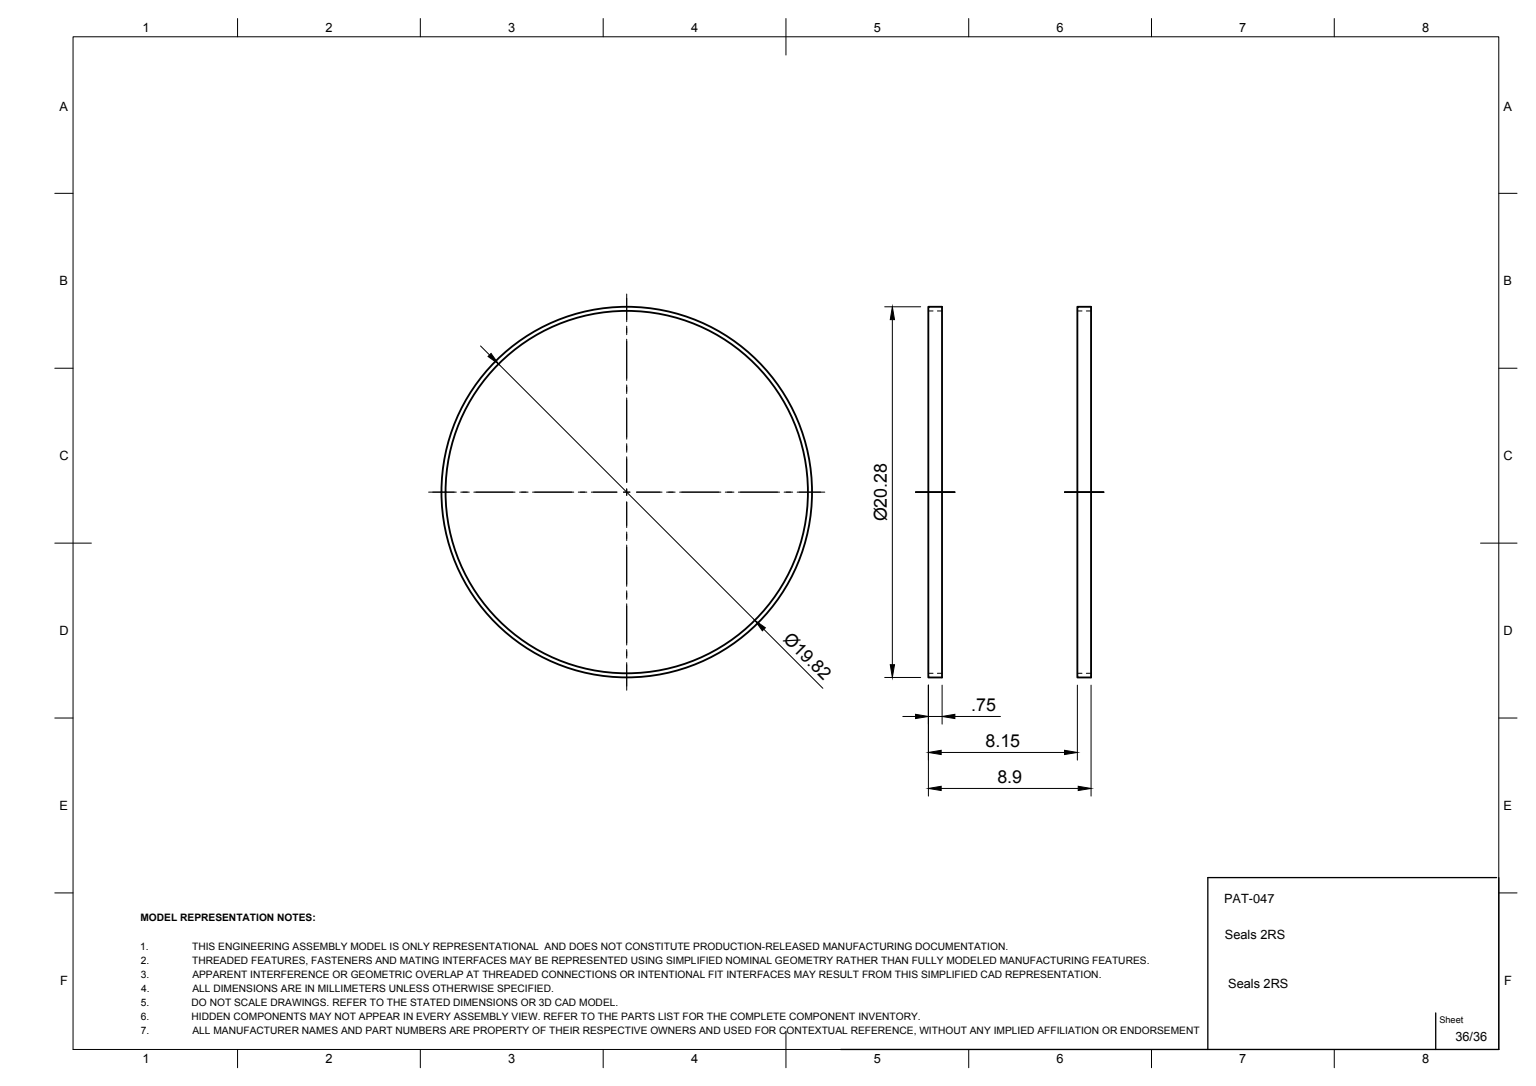
ISO-10303-21;
HEADER;
/* Generated by software containing ST-Developer
 * from STEP Tools, Inc. (www.steptools.com) 
 */

FILE_DESCRIPTION(
/* description */ ('Gravity roller conveyor section'),
/* implementation_level */ '2;1');

FILE_NAME(
/* name */ 'Seals 2RS.step',
/* time_stamp */ '2026-11-02T07:43:02-08:00',
/* author */ (''),
/* organization */ (''),
/* preprocessor_version */ 'ST-DEVELOPER v20.2',
/* originating_system */ 'Autodesk Translation Framework v15.17.0.0',
/* authorisation */ '');

FILE_SCHEMA (('AUTOMOTIVE_DESIGN { 1 0 10303 214 3 1 1 }'));
ENDSEC;

DATA;
#10=MECHANICAL_DESIGN_GEOMETRIC_PRESENTATION_REPRESENTATION('',(#563,#564),#13821);
#488=SHAPE_REPRESENTATION_RELATIONSHIP('SRR','None',#14027,#522);
#522=ADVANCED_BREP_SHAPE_REPRESENTATION('',(#603,#604),#13814);
#563=STYLED_ITEM('',(#14192),#603);
#564=STYLED_ITEM('',(#14192),#604);
#603=MANIFOLD_SOLID_BREP('Body1',#7663);
#604=MANIFOLD_SOLID_BREP('Body2',#7664);
#683=FACE_BOUND('',#1845,.T.);
#684=FACE_BOUND('',#1848,.T.);
#685=FACE_BOUND('',#1851,.T.);
#686=FACE_BOUND('',#1854,.T.);
#956=PLANE('',#8596);
#957=PLANE('',#8601);
#958=PLANE('',#8604);
#959=PLANE('',#8609);
#1351=FACE_OUTER_BOUND('',#1844,.T.);
#1352=FACE_OUTER_BOUND('',#1846,.T.);
#1353=FACE_OUTER_BOUND('',#1847,.T.);
#1354=FACE_OUTER_BOUND('',#1849,.T.);
#1355=FACE_OUTER_BOUND('',#1850,.T.);
#1356=FACE_OUTER_BOUND('',#1852,.T.);
#1357=FACE_OUTER_BOUND('',#1853,.T.);
#1358=FACE_OUTER_BOUND('',#1855,.T.);
#1844=EDGE_LOOP('',(#6830));
#1845=EDGE_LOOP('',(#6831));
#1846=EDGE_LOOP('',(#6832,#6833,#6834,#6835));
#1847=EDGE_LOOP('',(#6836));
#1848=EDGE_LOOP('',(#6837));
#1849=EDGE_LOOP('',(#6838,#6839,#6840,#6841));
#1850=EDGE_LOOP('',(#6842));
#1851=EDGE_LOOP('',(#6843));
#1852=EDGE_LOOP('',(#6844,#6845,#6846,#6847));
#1853=EDGE_LOOP('',(#6848));
#1854=EDGE_LOOP('',(#6849));
#1855=EDGE_LOOP('',(#6850,#6851,#6852,#6853));
#2552=LINE('',#13329,#3270);
#2553=LINE('',#13334,#3271);
#2554=LINE('',#13343,#3272);
#2555=LINE('',#13348,#3273);
#3270=VECTOR('',#10537,1.013815);
#3271=VECTOR('',#10544,0.991185);
#3272=VECTOR('',#10555,1.013815);
#3273=VECTOR('',#10562,0.991185);
#3546=CIRCLE('',#8597,1.013815);
#3547=CIRCLE('',#8598,0.991185);
#3548=CIRCLE('',#8600,1.013815);
#3549=CIRCLE('',#8602,0.991185);
#3550=CIRCLE('',#8605,1.013815);
#3551=CIRCLE('',#8606,0.991185);
#3552=CIRCLE('',#8608,1.013815);
#3553=CIRCLE('',#8610,0.991185);
#4140=VERTEX_POINT('',#13322);
#4141=VERTEX_POINT('',#13324);
#4142=VERTEX_POINT('',#13327);
#4143=VERTEX_POINT('',#13331);
#4144=VERTEX_POINT('',#13336);
#4145=VERTEX_POINT('',#13338);
#4146=VERTEX_POINT('',#13341);
#4147=VERTEX_POINT('',#13345);
#5052=EDGE_CURVE('',#4140,#4140,#3546,.T.);
#5053=EDGE_CURVE('',#4141,#4141,#3547,.T.);
#5054=EDGE_CURVE('',#4142,#4142,#3548,.T.);
#5055=EDGE_CURVE('',#4142,#4140,#2552,.T.);
#5056=EDGE_CURVE('',#4143,#4143,#3549,.T.);
#5057=EDGE_CURVE('',#4143,#4141,#2553,.T.);
#5058=EDGE_CURVE('',#4144,#4144,#3550,.T.);
#5059=EDGE_CURVE('',#4145,#4145,#3551,.T.);
#5060=EDGE_CURVE('',#4146,#4146,#3552,.T.);
#5061=EDGE_CURVE('',#4146,#4144,#2554,.T.);
#5062=EDGE_CURVE('',#4147,#4147,#3553,.T.);
#5063=EDGE_CURVE('',#4147,#4145,#2555,.T.);
#6830=ORIENTED_EDGE('',*,*,#5052,.F.);
#6831=ORIENTED_EDGE('',*,*,#5053,.T.);
#6832=ORIENTED_EDGE('',*,*,#5054,.F.);
#6833=ORIENTED_EDGE('',*,*,#5055,.T.);
#6834=ORIENTED_EDGE('',*,*,#5052,.T.);
#6835=ORIENTED_EDGE('',*,*,#5055,.F.);
#6836=ORIENTED_EDGE('',*,*,#5054,.T.);
#6837=ORIENTED_EDGE('',*,*,#5056,.F.);
#6838=ORIENTED_EDGE('',*,*,#5056,.T.);
#6839=ORIENTED_EDGE('',*,*,#5057,.T.);
#6840=ORIENTED_EDGE('',*,*,#5053,.F.);
#6841=ORIENTED_EDGE('',*,*,#5057,.F.);
#6842=ORIENTED_EDGE('',*,*,#5058,.F.);
#6843=ORIENTED_EDGE('',*,*,#5059,.T.);
#6844=ORIENTED_EDGE('',*,*,#5060,.F.);
#6845=ORIENTED_EDGE('',*,*,#5061,.T.);
#6846=ORIENTED_EDGE('',*,*,#5058,.T.);
#6847=ORIENTED_EDGE('',*,*,#5061,.F.);
#6848=ORIENTED_EDGE('',*,*,#5060,.T.);
#6849=ORIENTED_EDGE('',*,*,#5062,.F.);
#6850=ORIENTED_EDGE('',*,*,#5062,.T.);
#6851=ORIENTED_EDGE('',*,*,#5063,.T.);
#6852=ORIENTED_EDGE('',*,*,#5059,.F.);
#6853=ORIENTED_EDGE('',*,*,#5063,.F.);
#7190=CYLINDRICAL_SURFACE('',#8599,1.013815);
#7191=CYLINDRICAL_SURFACE('',#8603,0.991185);
#7192=CYLINDRICAL_SURFACE('',#8607,1.013815);
#7193=CYLINDRICAL_SURFACE('',#8611,0.991185);
#7552=ADVANCED_FACE('',(#1351,#683),#956,.T.);
#7553=ADVANCED_FACE('',(#1352),#7190,.T.);
#7554=ADVANCED_FACE('',(#1353,#684),#957,.T.);
#7555=ADVANCED_FACE('',(#1354),#7191,.F.);
#7556=ADVANCED_FACE('',(#1355,#685),#958,.T.);
#7557=ADVANCED_FACE('',(#1356),#7192,.T.);
#7558=ADVANCED_FACE('',(#1357,#686),#959,.T.);
#7559=ADVANCED_FACE('',(#1358),#7193,.F.);
#7663=CLOSED_SHELL('',(#7552,#7553,#7554,#7555));
#7664=CLOSED_SHELL('',(#7556,#7557,#7558,#7559));
#8595=AXIS2_PLACEMENT_3D('',#13320,#10525,#10526);
#8596=AXIS2_PLACEMENT_3D('',#13321,#10527,#10528);
#8597=AXIS2_PLACEMENT_3D('',#13323,#10529,#10530);
#8598=AXIS2_PLACEMENT_3D('',#13325,#10531,#10532);
#8599=AXIS2_PLACEMENT_3D('',#13326,#10533,#10534);
#8600=AXIS2_PLACEMENT_3D('',#13328,#10535,#10536);
#8601=AXIS2_PLACEMENT_3D('',#13330,#10538,#10539);
#8602=AXIS2_PLACEMENT_3D('',#13332,#10540,#10541);
#8603=AXIS2_PLACEMENT_3D('',#13333,#10542,#10543);
#8604=AXIS2_PLACEMENT_3D('',#13335,#10545,#10546);
#8605=AXIS2_PLACEMENT_3D('',#13337,#10547,#10548);
#8606=AXIS2_PLACEMENT_3D('',#13339,#10549,#10550);
#8607=AXIS2_PLACEMENT_3D('',#13340,#10551,#10552);
#8608=AXIS2_PLACEMENT_3D('',#13342,#10553,#10554);
#8609=AXIS2_PLACEMENT_3D('',#13344,#10556,#10557);
#8610=AXIS2_PLACEMENT_3D('',#13346,#10558,#10559);
#8611=AXIS2_PLACEMENT_3D('',#13347,#10560,#10561);
#10525=DIRECTION('axis',(0.,0.,1.));
#10526=DIRECTION('refdir',(1.,0.,0.));
#10527=DIRECTION('center_axis',(0.,1.,0.));
#10528=DIRECTION('ref_axis',(0.,0.,1.));
#10529=DIRECTION('center_axis',(0.,-1.,0.));
#10530=DIRECTION('ref_axis',(1.,0.,0.));
#10531=DIRECTION('center_axis',(0.,-1.,0.));
#10532=DIRECTION('ref_axis',(1.,0.,0.));
#10533=DIRECTION('center_axis',(0.,-1.,0.));
#10534=DIRECTION('ref_axis',(1.,0.,0.));
#10535=DIRECTION('center_axis',(0.,-1.,0.));
#10536=DIRECTION('ref_axis',(1.,0.,0.));
#10537=DIRECTION('',(0.,1.,0.));
#10538=DIRECTION('center_axis',(0.,-1.,0.));
#10539=DIRECTION('ref_axis',(0.,0.,-1.));
#10540=DIRECTION('center_axis',(0.,-1.,0.));
#10541=DIRECTION('ref_axis',(1.,0.,0.));
#10542=DIRECTION('center_axis',(0.,-1.,0.));
#10543=DIRECTION('ref_axis',(1.,0.,0.));
#10544=DIRECTION('',(0.,1.,0.));
#10545=DIRECTION('center_axis',(0.,1.,0.));
#10546=DIRECTION('ref_axis',(0.,0.,1.));
#10547=DIRECTION('center_axis',(0.,-1.,0.));
#10548=DIRECTION('ref_axis',(1.,0.,0.));
#10549=DIRECTION('center_axis',(0.,-1.,0.));
#10550=DIRECTION('ref_axis',(1.,0.,0.));
#10551=DIRECTION('center_axis',(0.,-1.,0.));
#10552=DIRECTION('ref_axis',(1.,0.,0.));
#10553=DIRECTION('center_axis',(0.,-1.,0.));
#10554=DIRECTION('ref_axis',(1.,0.,0.));
#10555=DIRECTION('',(0.,1.,0.));
#10556=DIRECTION('center_axis',(0.,-1.,0.));
#10557=DIRECTION('ref_axis',(0.,0.,-1.));
#10558=DIRECTION('center_axis',(0.,-1.,0.));
#10559=DIRECTION('ref_axis',(1.,0.,0.));
#10560=DIRECTION('center_axis',(0.,-1.,0.));
#10561=DIRECTION('ref_axis',(1.,0.,0.));
#10562=DIRECTION('',(0.,1.,0.));
#13320=CARTESIAN_POINT('',(0.,0.,0.));
#13321=CARTESIAN_POINT('Origin',(1.013815,0.445,0.));
#13322=CARTESIAN_POINT('',(-1.013815,0.445,-1.24156529467757E-16));
#13323=CARTESIAN_POINT('Origin',(0.,0.445,0.));
#13324=CARTESIAN_POINT('',(-0.991185,0.445,-1.21385153761287E-16));
#13325=CARTESIAN_POINT('Origin',(0.,0.445,0.));
#13326=CARTESIAN_POINT('Origin',(0.,0.4075,0.));
#13327=CARTESIAN_POINT('',(-1.013815,0.37,-1.24156529467757E-16));
#13328=CARTESIAN_POINT('Origin',(0.,0.37,0.));
#13329=CARTESIAN_POINT('',(-1.013815,0.4075,-1.24156529467757E-16));
#13330=CARTESIAN_POINT('Origin',(0.991185,0.37,0.));
#13331=CARTESIAN_POINT('',(-0.991185,0.37,-1.21385153761287E-16));
#13332=CARTESIAN_POINT('Origin',(0.,0.37,0.));
#13333=CARTESIAN_POINT('Origin',(0.,0.4075,0.));
#13334=CARTESIAN_POINT('',(-0.991185,0.4075,-1.21385153761287E-16));
#13335=CARTESIAN_POINT('Origin',(1.013815,-0.37,0.));
#13336=CARTESIAN_POINT('',(-1.013815,-0.37,-1.24156529467757E-16));
#13337=CARTESIAN_POINT('Origin',(0.,-0.37,0.));
#13338=CARTESIAN_POINT('',(-0.991185,-0.37,-1.21385153761287E-16));
#13339=CARTESIAN_POINT('Origin',(0.,-0.37,0.));
#13340=CARTESIAN_POINT('Origin',(0.,-0.4075,0.));
#13341=CARTESIAN_POINT('',(-1.013815,-0.445,-1.24156529467757E-16));
#13342=CARTESIAN_POINT('Origin',(0.,-0.445,0.));
#13343=CARTESIAN_POINT('',(-1.013815,-0.4075,-1.24156529467757E-16));
#13344=CARTESIAN_POINT('Origin',(0.991185,-0.445,0.));
#13345=CARTESIAN_POINT('',(-0.991185,-0.445,-1.21385153761287E-16));
#13346=CARTESIAN_POINT('Origin',(0.,-0.445,0.));
#13347=CARTESIAN_POINT('Origin',(0.,-0.4075,0.));
#13348=CARTESIAN_POINT('',(-0.991185,-0.4075,-1.21385153761287E-16));
#13775=UNCERTAINTY_MEASURE_WITH_UNIT(LENGTH_MEASURE(0.001),#13822,
'DISTANCE_ACCURACY_VALUE',
'Maximum model space distance between geometric entities at asserted c
onnectivities');
#13782=UNCERTAINTY_MEASURE_WITH_UNIT(LENGTH_MEASURE(0.001),#13822,
'DISTANCE_ACCURACY_VALUE',
'Maximum model space distance between geometric entities at asserted c
onnectivities');
#13814=(
GEOMETRIC_REPRESENTATION_CONTEXT(3)
GLOBAL_UNCERTAINTY_ASSIGNED_CONTEXT((#13775))
GLOBAL_UNIT_ASSIGNED_CONTEXT((#13822,#13824,#13825))
REPRESENTATION_CONTEXT('','3D')
);
#13821=(
GEOMETRIC_REPRESENTATION_CONTEXT(3)
GLOBAL_UNCERTAINTY_ASSIGNED_CONTEXT((#13782))
GLOBAL_UNIT_ASSIGNED_CONTEXT((#13822,#13824,#13825))
REPRESENTATION_CONTEXT('','3D')
);
#13822=(
LENGTH_UNIT()
NAMED_UNIT(*)
SI_UNIT(.CENTI.,.METRE.)
);
#13824=(
NAMED_UNIT(*)
PLANE_ANGLE_UNIT()
SI_UNIT($,.RADIAN.)
);
#13825=(
NAMED_UNIT(*)
SI_UNIT($,.STERADIAN.)
SOLID_ANGLE_UNIT()
);
#13857=SHAPE_DEFINITION_REPRESENTATION(#13895,#14027);
#13895=PRODUCT_DEFINITION_SHAPE('',$,#14066);
#14027=SHAPE_REPRESENTATION('',(#8595),#13814);
#14034=PRODUCT_DEFINITION_CONTEXT('part definition',#14150,'design');
#14066=PRODUCT_DEFINITION('Seals 2RS','Seals 2RS',#14104,#14034);
#14104=PRODUCT_DEFINITION_FORMATION('',$,#14183);
#14150=APPLICATION_CONTEXT(
'Core Data for Automotive Mechanical Design Process');
#14151=PRODUCT_CONTEXT('part definition',#14150,'mechanical');
#14183=PRODUCT('Seals 2RS','Seals 2RS','Seals 2RS',(#14151));
#14192=PRESENTATION_STYLE_ASSIGNMENT((#14197));
#14197=SURFACE_STYLE_USAGE(.BOTH.,#14202);
#14202=SURFACE_SIDE_STYLE('',(#14207));
#14207=SURFACE_STYLE_FILL_AREA(#14212);
#14212=FILL_AREA_STYLE('CAD Library Painted - Engineering blue',(#14217));
#14217=FILL_AREA_STYLE_COLOUR('CAD Library Painted - Engineering blue',
#14222);
#14222=COLOUR_RGB('CAD Library Painted - Engineering blue',0.12156862745098,
0.356862745098039,0.6);
ENDSEC;
END-ISO-10303-21;
